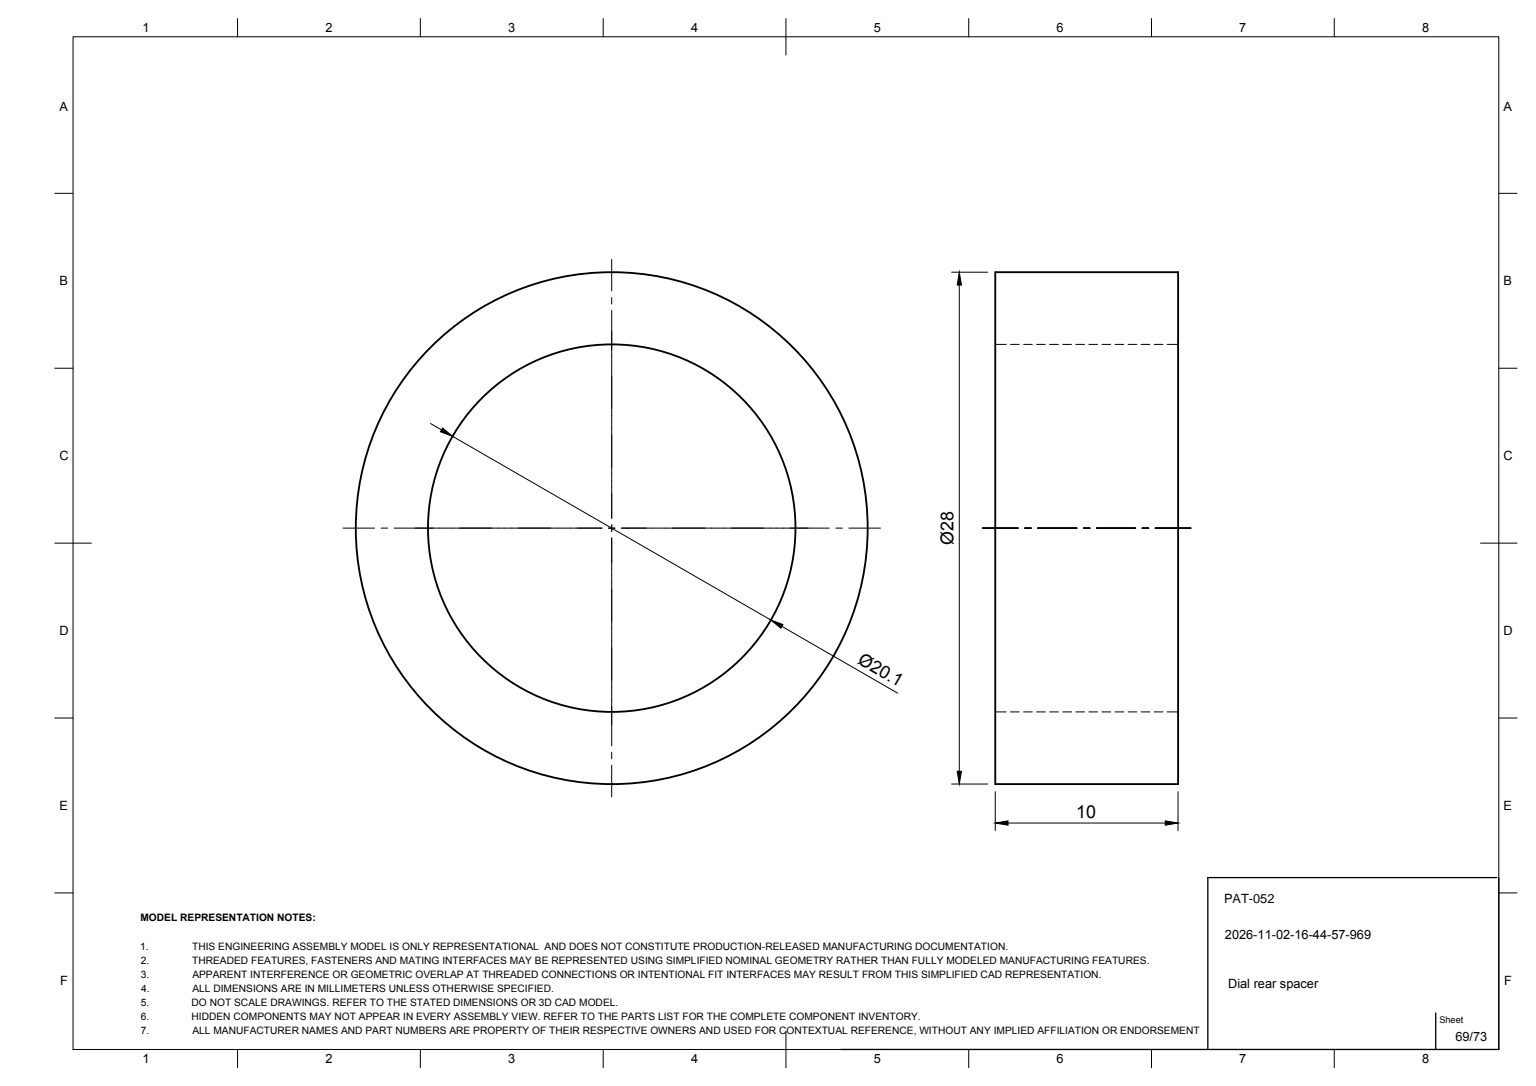
ISO-10303-21;
HEADER;
/* Generated by software containing ST-Developer
 * from STEP Tools, Inc. (www.steptools.com) 
 */

FILE_DESCRIPTION(
/* description */ ('Hand-crank gear train demonstrator'),
/* implementation_level */ '2;1');

FILE_NAME(
/* name */ 'Dial rear spacer.step',
/* time_stamp */ '2026-10-28T03:22:13-07:00',
/* author */ (''),
/* organization */ (''),
/* preprocessor_version */ 'ST-DEVELOPER v20.2',
/* originating_system */ 'Autodesk Translation Framework v15.17.0.0',
/* authorisation */ '');

FILE_SCHEMA (('AUTOMOTIVE_DESIGN { 1 0 10303 214 3 1 1 }'));
ENDSEC;

DATA;
#10=MECHANICAL_DESIGN_GEOMETRIC_PRESENTATION_REPRESENTATION('',(#1259),#62758);
#1116=SHAPE_REPRESENTATION_RELATIONSHIP('SRR','None',#63094,#1180);
#1180=ADVANCED_BREP_SHAPE_REPRESENTATION('',(#1334),#62748);
#1259=STYLED_ITEM('',(#63455),#1334);
#1334=MANIFOLD_SOLID_BREP('Body1',#16443);
#1615=FACE_BOUND('',#4037,.T.);
#1616=FACE_BOUND('',#4039,.T.);
#2031=PLANE('',#18441);
#2032=PLANE('',#18442);
#2825=FACE_OUTER_BOUND('',#4034,.T.);
#2826=FACE_OUTER_BOUND('',#4035,.T.);
#2827=FACE_OUTER_BOUND('',#4036,.T.);
#2828=FACE_OUTER_BOUND('',#4038,.T.);
#4034=EDGE_LOOP('',(#13917,#13918,#13919,#13920));
#4035=EDGE_LOOP('',(#13921,#13922,#13923,#13924));
#4036=EDGE_LOOP('',(#13925));
#4037=EDGE_LOOP('',(#13926));
#4038=EDGE_LOOP('',(#13927));
#4039=EDGE_LOOP('',(#13928));
#5158=LINE('',#38608,#6290);
#5159=LINE('',#38614,#6291);
#6290=VECTOR('',#22261,1.005);
#6291=VECTOR('',#22268,1.4);
#7091=CIRCLE('',#18436,1.005);
#7092=CIRCLE('',#18437,1.005);
#7093=CIRCLE('',#18439,1.4);
#7094=CIRCLE('',#18440,1.4);
#8254=VERTEX_POINT('',#38605);
#8255=VERTEX_POINT('',#38607);
#8256=VERTEX_POINT('',#38611);
#8257=VERTEX_POINT('',#38613);
#10210=EDGE_CURVE('',#8254,#8254,#7091,.T.);
#10211=EDGE_CURVE('',#8254,#8255,#5158,.T.);
#10212=EDGE_CURVE('',#8255,#8255,#7092,.T.);
#10213=EDGE_CURVE('',#8256,#8256,#7093,.T.);
#10214=EDGE_CURVE('',#8256,#8257,#5159,.T.);
#10215=EDGE_CURVE('',#8257,#8257,#7094,.T.);
#13917=ORIENTED_EDGE('',*,*,#10210,.F.);
#13918=ORIENTED_EDGE('',*,*,#10211,.T.);
#13919=ORIENTED_EDGE('',*,*,#10212,.T.);
#13920=ORIENTED_EDGE('',*,*,#10211,.F.);
#13921=ORIENTED_EDGE('',*,*,#10213,.F.);
#13922=ORIENTED_EDGE('',*,*,#10214,.T.);
#13923=ORIENTED_EDGE('',*,*,#10215,.T.);
#13924=ORIENTED_EDGE('',*,*,#10214,.F.);
#13925=ORIENTED_EDGE('',*,*,#10213,.T.);
#13926=ORIENTED_EDGE('',*,*,#10210,.T.);
#13927=ORIENTED_EDGE('',*,*,#10215,.F.);
#13928=ORIENTED_EDGE('',*,*,#10212,.F.);
#15377=CYLINDRICAL_SURFACE('',#18435,1.005);
#15378=CYLINDRICAL_SURFACE('',#18438,1.4);
#16135=ADVANCED_FACE('',(#2825),#15377,.F.);
#16136=ADVANCED_FACE('',(#2826),#15378,.T.);
#16137=ADVANCED_FACE('',(#2827,#1615),#2031,.T.);
#16138=ADVANCED_FACE('',(#2828,#1616),#2032,.F.);
#16443=CLOSED_SHELL('',(#16135,#16136,#16137,#16138));
#18434=AXIS2_PLACEMENT_3D('',#38603,#22255,#22256);
#18435=AXIS2_PLACEMENT_3D('',#38604,#22257,#22258);
#18436=AXIS2_PLACEMENT_3D('',#38606,#22259,#22260);
#18437=AXIS2_PLACEMENT_3D('',#38609,#22262,#22263);
#18438=AXIS2_PLACEMENT_3D('',#38610,#22264,#22265);
#18439=AXIS2_PLACEMENT_3D('',#38612,#22266,#22267);
#18440=AXIS2_PLACEMENT_3D('',#38615,#22269,#22270);
#18441=AXIS2_PLACEMENT_3D('',#38616,#22271,#22272);
#18442=AXIS2_PLACEMENT_3D('',#38617,#22273,#22274);
#22255=DIRECTION('axis',(0.,0.,1.));
#22256=DIRECTION('refdir',(1.,0.,0.));
#22257=DIRECTION('center_axis',(0.,1.,0.));
#22258=DIRECTION('ref_axis',(1.,0.,0.));
#22259=DIRECTION('center_axis',(0.,-1.,0.));
#22260=DIRECTION('ref_axis',(1.,0.,0.));
#22261=DIRECTION('',(0.,-1.,0.));
#22262=DIRECTION('center_axis',(0.,-1.,0.));
#22263=DIRECTION('ref_axis',(1.,0.,0.));
#22264=DIRECTION('center_axis',(0.,1.,0.));
#22265=DIRECTION('ref_axis',(1.,0.,0.));
#22266=DIRECTION('center_axis',(0.,1.,0.));
#22267=DIRECTION('ref_axis',(1.,0.,0.));
#22268=DIRECTION('',(0.,-1.,0.));
#22269=DIRECTION('center_axis',(0.,1.,0.));
#22270=DIRECTION('ref_axis',(1.,0.,0.));
#22271=DIRECTION('center_axis',(0.,1.,0.));
#22272=DIRECTION('ref_axis',(1.,0.,0.));
#22273=DIRECTION('center_axis',(0.,1.,0.));
#22274=DIRECTION('ref_axis',(1.,0.,0.));
#38603=CARTESIAN_POINT('',(0.,0.,0.));
#38604=CARTESIAN_POINT('Origin',(18.,3.2,9.));
#38605=CARTESIAN_POINT('',(16.995,4.2,9.));
#38606=CARTESIAN_POINT('Origin',(18.,4.2,9.));
#38607=CARTESIAN_POINT('',(16.995,3.2,9.));
#38608=CARTESIAN_POINT('',(16.995,3.2,9.));
#38609=CARTESIAN_POINT('Origin',(18.,3.2,9.));
#38610=CARTESIAN_POINT('Origin',(18.,3.2,9.));
#38611=CARTESIAN_POINT('',(16.6,4.2,9.));
#38612=CARTESIAN_POINT('Origin',(18.,4.2,9.));
#38613=CARTESIAN_POINT('',(16.6,3.2,9.));
#38614=CARTESIAN_POINT('',(16.6,3.2,9.));
#38615=CARTESIAN_POINT('Origin',(18.,3.2,9.));
#38616=CARTESIAN_POINT('Origin',(18.,4.2,9.));
#38617=CARTESIAN_POINT('Origin',(18.,3.2,9.));
#62674=UNCERTAINTY_MEASURE_WITH_UNIT(LENGTH_MEASURE(0.001),#62759,
'DISTANCE_ACCURACY_VALUE',
'Maximum model space distance between geometric entities at asserted c
onnectivities');
#62684=UNCERTAINTY_MEASURE_WITH_UNIT(LENGTH_MEASURE(0.001),#62759,
'DISTANCE_ACCURACY_VALUE',
'Maximum model space distance between geometric entities at asserted c
onnectivities');
#62748=(
GEOMETRIC_REPRESENTATION_CONTEXT(3)
GLOBAL_UNCERTAINTY_ASSIGNED_CONTEXT((#62674))
GLOBAL_UNIT_ASSIGNED_CONTEXT((#62759,#62761,#62762))
REPRESENTATION_CONTEXT('','3D')
);
#62758=(
GEOMETRIC_REPRESENTATION_CONTEXT(3)
GLOBAL_UNCERTAINTY_ASSIGNED_CONTEXT((#62684))
GLOBAL_UNIT_ASSIGNED_CONTEXT((#62759,#62761,#62762))
REPRESENTATION_CONTEXT('','3D')
);
#62759=(
LENGTH_UNIT()
NAMED_UNIT(*)
SI_UNIT(.CENTI.,.METRE.)
);
#62761=(
NAMED_UNIT(*)
PLANE_ANGLE_UNIT()
SI_UNIT($,.RADIAN.)
);
#62762=(
NAMED_UNIT(*)
SI_UNIT($,.STERADIAN.)
SOLID_ANGLE_UNIT()
);
#62826=SHAPE_DEFINITION_REPRESENTATION(#62909,#63094);
#62909=PRODUCT_DEFINITION_SHAPE('',$,#63168);
#63094=SHAPE_REPRESENTATION('',(#18434),#62748);
#63104=PRODUCT_DEFINITION_CONTEXT('part definition',#63325,'design');
#63168=PRODUCT_DEFINITION('Dial rear spacer','Dial rear spacer',#63241,
#63104);
#63241=PRODUCT_DEFINITION_FORMATION('',$,#63390);
#63325=APPLICATION_CONTEXT(
'Core Data for Automotive Mechanical Design Process');
#63326=PRODUCT_CONTEXT('part definition',#63325,'mechanical');
#63390=PRODUCT('Dial rear spacer','Dial rear spacer','Dial rear spacer',
(#63326));
#63449=COLOUR_RGB('Sky Blue',0.24,0.69,0.87);
#63450=FILL_AREA_STYLE_COLOUR('',#63449);
#63451=FILL_AREA_STYLE('',(#63450));
#63452=SURFACE_STYLE_FILL_AREA(#63451);
#63453=SURFACE_SIDE_STYLE('',(#63452));
#63454=SURFACE_STYLE_USAGE(.BOTH.,#63453);
#63455=PRESENTATION_STYLE_ASSIGNMENT((#63454));
ENDSEC;
END-ISO-10303-21;
